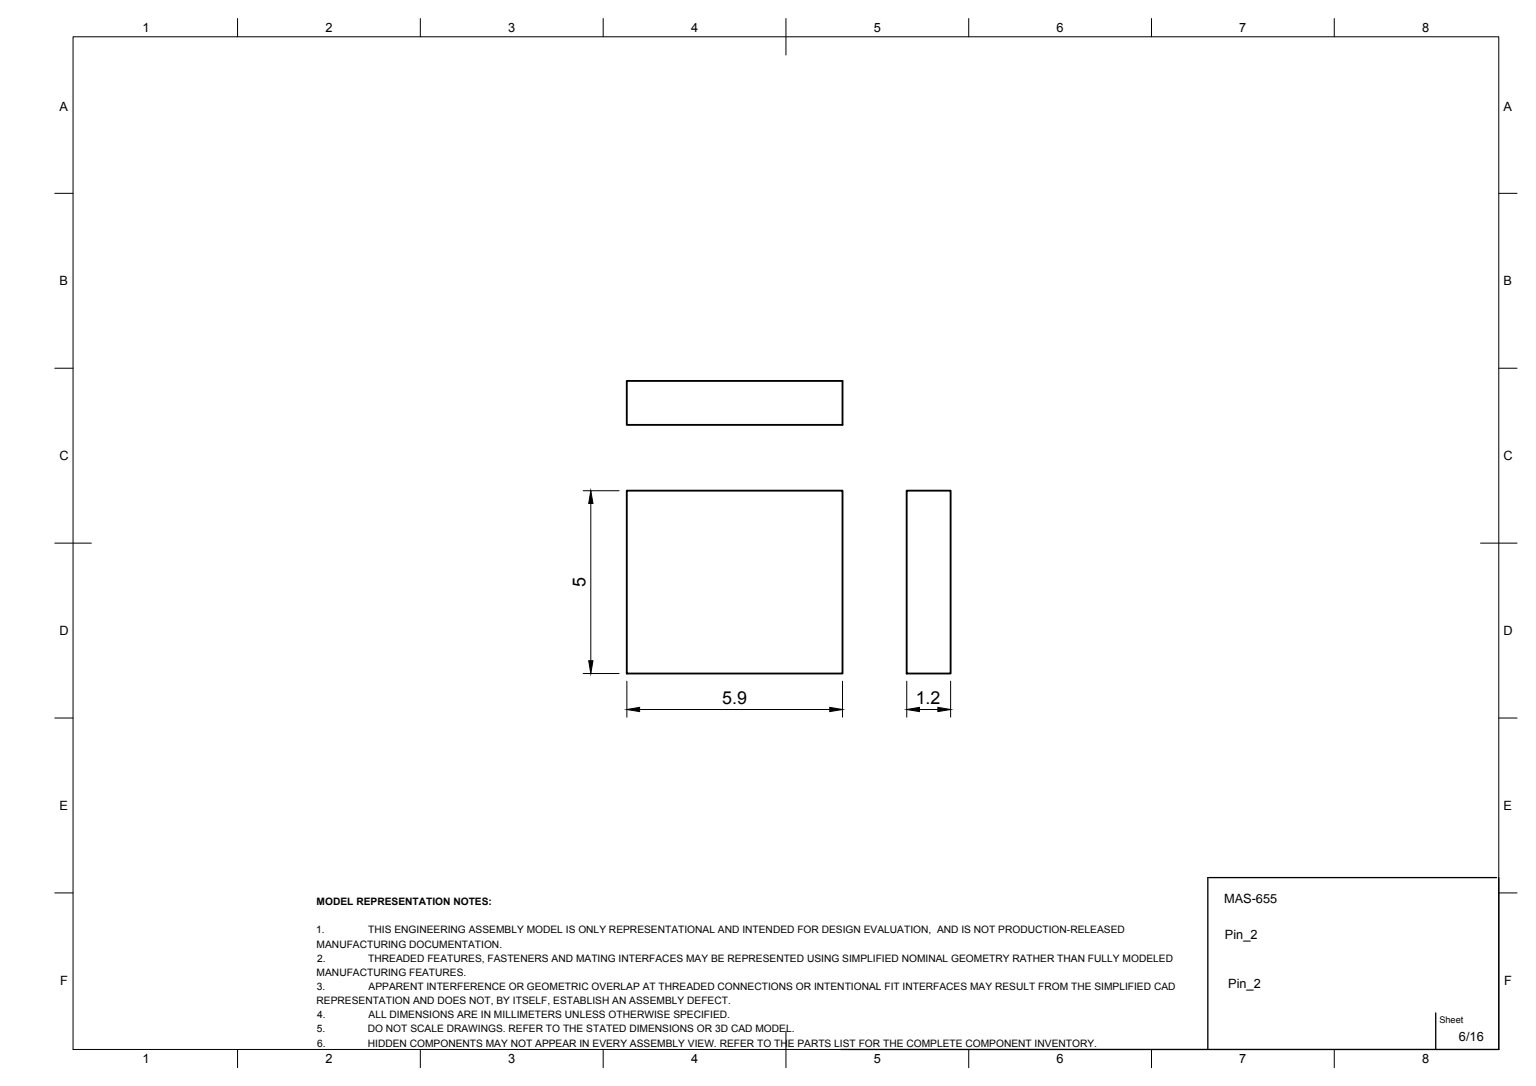
ISO-10303-21;
HEADER;
FILE_DESCRIPTION((''),'2;1');
FILE_NAME('Pin_2.step','2026-10-09T11:34:15-07:00',(''),(''),'','','');
FILE_SCHEMA (('AUTOMOTIVE_DESIGN { 1 0 10303 214 3 1 1 }'));
ENDSEC;
DATA;
#10=MECHANICAL_DESIGN_GEOMETRIC_PRESENTATION_REPRESENTATION('',(#633),#117170);
#591=SHAPE_REPRESENTATION_RELATIONSHIP('SRR','None',#117246,#612) ;
#612=ADVANCED_BREP_SHAPE_REPRESENTATION('',(#654),#117154) ;
#633=STYLED_ITEM('',(#117355),#654) ;
#654=MANIFOLD_SOLID_BREP('Body1',#49062) ;
#2476=PLANE('',#51975) ;
#2477=PLANE('',#51976) ;
#2478=PLANE('',#51977) ;
#2479=PLANE('',#51978) ;
#2480=PLANE('',#51979) ;
#2481=PLANE('',#51980) ;
#4253=LINE('',#87449,#7467) ;
#4254=LINE('',#87451,#7468) ;
#4255=LINE('',#87453,#7469) ;
#4256=LINE('',#87454,#7470) ;
#4257=LINE('',#87457,#7471) ;
#4258=LINE('',#87459,#7472) ;
#4259=LINE('',#87460,#7473) ;
#4260=LINE('',#87463,#7474) ;
#4261=LINE('',#87465,#7475) ;
#4262=LINE('',#87466,#7476) ;
#4263=LINE('',#87468,#7477) ;
#4264=LINE('',#87469,#7478) ;
#7467=VECTOR('',#61650,10.) ;
#7468=VECTOR('',#61651,10.) ;
#7469=VECTOR('',#61652,10.) ;
#7470=VECTOR('',#61653,10.) ;
#7471=VECTOR('',#61656,10.) ;
#7472=VECTOR('',#61657,10.) ;
#7473=VECTOR('',#61658,10.) ;
#7474=VECTOR('',#61661,10.) ;
#7475=VECTOR('',#61662,10.) ;
#7476=VECTOR('',#61663,10.) ;
#7477=VECTOR('',#61666,10.) ;
#7478=VECTOR('',#61667,10.) ;
#12097=FACE_OUTER_BOUND('',#15248,.T.) ;
#12098=FACE_OUTER_BOUND('',#15249,.T.) ;
#12099=FACE_OUTER_BOUND('',#15250,.T.) ;
#12100=FACE_OUTER_BOUND('',#15251,.T.) ;
#12101=FACE_OUTER_BOUND('',#15252,.T.) ;
#12102=FACE_OUTER_BOUND('',#15253,.T.) ;
#15248=EDGE_LOOP('',(#37250,#37251,#37252,#37253)) ;
#15249=EDGE_LOOP('',(#37254,#37255,#37256,#37257)) ;
#15250=EDGE_LOOP('',(#37258,#37259,#37260,#37261)) ;
#15251=EDGE_LOOP('',(#37262,#37263,#37264,#37265)) ;
#15252=EDGE_LOOP('',(#37266,#37267,#37268,#37269)) ;
#15253=EDGE_LOOP('',(#37270,#37271,#37272,#37273)) ;
#21368=VERTEX_POINT('',#87447) ;
#21369=VERTEX_POINT('',#87448) ;
#21370=VERTEX_POINT('',#87450) ;
#21371=VERTEX_POINT('',#87452) ;
#21372=VERTEX_POINT('',#87456) ;
#21373=VERTEX_POINT('',#87458) ;
#21374=VERTEX_POINT('',#87462) ;
#21375=VERTEX_POINT('',#87464) ;
#26903=EDGE_CURVE('',#21368,#21369,#4253,.T.) ;
#26904=EDGE_CURVE('',#21369,#21370,#4254,.T.) ;
#26905=EDGE_CURVE('',#21371,#21370,#4255,.T.) ;
#26906=EDGE_CURVE('',#21368,#21371,#4256,.T.) ;
#26907=EDGE_CURVE('',#21372,#21368,#4257,.T.) ;
#26908=EDGE_CURVE('',#21373,#21371,#4258,.T.) ;
#26909=EDGE_CURVE('',#21372,#21373,#4259,.T.) ;
#26910=EDGE_CURVE('',#21374,#21372,#4260,.T.) ;
#26911=EDGE_CURVE('',#21375,#21373,#4261,.T.) ;
#26912=EDGE_CURVE('',#21374,#21375,#4262,.T.) ;
#26913=EDGE_CURVE('',#21369,#21374,#4263,.T.) ;
#26914=EDGE_CURVE('',#21370,#21375,#4264,.T.) ;
#37250=ORIENTED_EDGE('',*,*,#26903,.T.) ;
#37251=ORIENTED_EDGE('',*,*,#26904,.T.) ;
#37252=ORIENTED_EDGE('',*,*,#26905,.F.) ;
#37253=ORIENTED_EDGE('',*,*,#26906,.F.) ;
#37254=ORIENTED_EDGE('',*,*,#26907,.T.) ;
#37255=ORIENTED_EDGE('',*,*,#26906,.T.) ;
#37256=ORIENTED_EDGE('',*,*,#26908,.F.) ;
#37257=ORIENTED_EDGE('',*,*,#26909,.F.) ;
#37258=ORIENTED_EDGE('',*,*,#26910,.T.) ;
#37259=ORIENTED_EDGE('',*,*,#26909,.T.) ;
#37260=ORIENTED_EDGE('',*,*,#26911,.F.) ;
#37261=ORIENTED_EDGE('',*,*,#26912,.F.) ;
#37262=ORIENTED_EDGE('',*,*,#26913,.T.) ;
#37263=ORIENTED_EDGE('',*,*,#26912,.T.) ;
#37264=ORIENTED_EDGE('',*,*,#26914,.F.) ;
#37265=ORIENTED_EDGE('',*,*,#26904,.F.) ;
#37266=ORIENTED_EDGE('',*,*,#26914,.T.) ;
#37267=ORIENTED_EDGE('',*,*,#26911,.T.) ;
#37268=ORIENTED_EDGE('',*,*,#26908,.T.) ;
#37269=ORIENTED_EDGE('',*,*,#26905,.T.) ;
#37270=ORIENTED_EDGE('',*,*,#26913,.F.) ;
#37271=ORIENTED_EDGE('',*,*,#26903,.F.) ;
#37272=ORIENTED_EDGE('',*,*,#26907,.F.) ;
#37273=ORIENTED_EDGE('',*,*,#26910,.F.) ;
#47315=ADVANCED_FACE('',(#12097),#2476,.T.) ;
#47316=ADVANCED_FACE('',(#12098),#2477,.T.) ;
#47317=ADVANCED_FACE('',(#12099),#2478,.T.) ;
#47318=ADVANCED_FACE('',(#12100),#2479,.T.) ;
#47319=ADVANCED_FACE('',(#12101),#2480,.T.) ;
#47320=ADVANCED_FACE('',(#12102),#2481,.F.) ;
#49062=CLOSED_SHELL('',(#47315,#47316,#47317,#47318,#47319,#47320)) ;
#51974=AXIS2_PLACEMENT_3D('',#87445,#61646,#61647) ;
#51975=AXIS2_PLACEMENT_3D('',#87446,#61648,#61649) ;
#51976=AXIS2_PLACEMENT_3D('',#87455,#61654,#61655) ;
#51977=AXIS2_PLACEMENT_3D('',#87461,#61659,#61660) ;
#51978=AXIS2_PLACEMENT_3D('',#87467,#61664,#61665) ;
#51979=AXIS2_PLACEMENT_3D('',#87470,#61668,#61669) ;
#51980=AXIS2_PLACEMENT_3D('',#87471,#61670,#61671) ;
#61646=DIRECTION('axis',(0.,0.,1.)) ;
#61647=DIRECTION('refdir',(1.,0.,0.)) ;
#61648=DIRECTION('center_axis',(0.,-1.,0.)) ;
#61649=DIRECTION('ref_axis',(-1.,0.,-2.52374105052742E-18)) ;
#61650=DIRECTION('',(-1.,0.,-2.52374105052742E-18)) ;
#61651=DIRECTION('',(0.,0.,-1.)) ;
#61652=DIRECTION('',(-1.,0.,-2.52374105052742E-18)) ;
#61653=DIRECTION('',(0.,0.,-1.)) ;
#61654=DIRECTION('center_axis',(1.,1.41426179436738E-51,0.)) ;
#61655=DIRECTION('ref_axis',(1.41426179436738E-51,-1.,-5.60383084497445E-34)) ;
#61656=DIRECTION('',(1.41426179436738E-51,-1.,-5.60383084497445E-34)) ;
#61657=DIRECTION('',(1.41426179436738E-51,-1.,-5.60383084497445E-34)) ;
#61658=DIRECTION('',(0.,0.,-1.)) ;
#61659=DIRECTION('center_axis',(0.,1.,0.)) ;
#61660=DIRECTION('ref_axis',(1.,0.,2.52374105052742E-18)) ;
#61661=DIRECTION('',(1.,0.,2.52374105052742E-18)) ;
#61662=DIRECTION('',(1.,0.,2.52374105052742E-18)) ;
#61663=DIRECTION('',(0.,0.,-1.)) ;
#61664=DIRECTION('center_axis',(-1.,-1.41426179436738E-51,0.)) ;
#61665=DIRECTION('ref_axis',(-1.41426179436738E-51,1.,5.60383084497445E-34)) ;
#61666=DIRECTION('',(-1.41426179436738E-51,1.,5.60383084497445E-34)) ;
#61667=DIRECTION('',(-1.41426179436738E-51,1.,5.60383084497445E-34)) ;
#61668=DIRECTION('center_axis',(0.,0.,-1.)) ;
#61669=DIRECTION('ref_axis',(-1.,0.,0.)) ;
#61670=DIRECTION('center_axis',(2.52374105052742E-18,5.60383084497445E-34,
-1.)) ;
#61671=DIRECTION('ref_axis',(1.,3.40207761657885E-68,2.52374105052742E-18)) ;
#87445=CARTESIAN_POINT('',(0.,0.,0.)) ;
#87446=CARTESIAN_POINT('Origin',(34.2,257.9,30.7213203435596)) ;
#87447=CARTESIAN_POINT('',(34.2,257.9,30.7213203435596)) ;
#87448=CARTESIAN_POINT('',(29.2,257.9,30.7213203435596)) ;
#87449=CARTESIAN_POINT('',(34.2,257.9,30.7213203435596)) ;
#87450=CARTESIAN_POINT('',(29.2,257.9,29.5213203435596)) ;
#87451=CARTESIAN_POINT('',(29.2,257.9,30.7213203435596)) ;
#87452=CARTESIAN_POINT('',(34.2,257.9,29.5213203435596)) ;
#87453=CARTESIAN_POINT('',(34.2,257.9,29.5213203435596)) ;
#87454=CARTESIAN_POINT('',(34.2,257.9,30.7213203435596)) ;
#87455=CARTESIAN_POINT('Origin',(34.2,263.8,30.7213203435596)) ;
#87456=CARTESIAN_POINT('',(34.2,263.8,30.7213203435596)) ;
#87457=CARTESIAN_POINT('',(34.2,263.8,30.7213203435596)) ;
#87458=CARTESIAN_POINT('',(34.2,263.8,29.5213203435596)) ;
#87459=CARTESIAN_POINT('',(34.2,263.8,29.5213203435596)) ;
#87460=CARTESIAN_POINT('',(34.2,263.8,30.7213203435596)) ;
#87461=CARTESIAN_POINT('Origin',(29.2,263.8,30.7213203435596)) ;
#87462=CARTESIAN_POINT('',(29.2,263.8,30.7213203435596)) ;
#87463=CARTESIAN_POINT('',(29.2,263.8,30.7213203435596)) ;
#87464=CARTESIAN_POINT('',(29.2,263.8,29.5213203435596)) ;
#87465=CARTESIAN_POINT('',(29.2,263.8,29.5213203435596)) ;
#87466=CARTESIAN_POINT('',(29.2,263.8,30.7213203435596)) ;
#87467=CARTESIAN_POINT('Origin',(29.2,257.9,30.7213203435596)) ;
#87468=CARTESIAN_POINT('',(29.2,257.9,30.7213203435596)) ;
#87469=CARTESIAN_POINT('',(29.2,257.9,29.5213203435596)) ;
#87470=CARTESIAN_POINT('Origin',(31.7,260.85,29.5213203435596)) ;
#87471=CARTESIAN_POINT('Origin',(31.7,260.85,30.7213203435596)) ;
#117131=UNCERTAINTY_MEASURE_WITH_UNIT(LENGTH_MEASURE(0.01),#117171,
'DISTANCE_ACCURACY_VALUE',
'Maximum model space distance between geometric entities at asserted c
onnectivities') ;
#117147=UNCERTAINTY_MEASURE_WITH_UNIT(LENGTH_MEASURE(0.01),#117171,
'DISTANCE_ACCURACY_VALUE',
'Maximum model space distance between geometric entities at asserted c
onnectivities') ;
#117154=(
GEOMETRIC_REPRESENTATION_CONTEXT(3)
GLOBAL_UNCERTAINTY_ASSIGNED_CONTEXT((#117131))
GLOBAL_UNIT_ASSIGNED_CONTEXT((#117171,#117173,#117174))
REPRESENTATION_CONTEXT('','3D')
) ;
#117170=(
GEOMETRIC_REPRESENTATION_CONTEXT(3)
GLOBAL_UNCERTAINTY_ASSIGNED_CONTEXT((#117147))
GLOBAL_UNIT_ASSIGNED_CONTEXT((#117171,#117173,#117174))
REPRESENTATION_CONTEXT('','3D')
) ;
#117171=(
LENGTH_UNIT()
NAMED_UNIT(*)
SI_UNIT(.MILLI.,.METRE.)
) ;
#117173=(
NAMED_UNIT(*)
PLANE_ANGLE_UNIT()
SI_UNIT($,.RADIAN.)
) ;
#117174=(
NAMED_UNIT(*)
SI_UNIT($,.STERADIAN.)
SOLID_ANGLE_UNIT()
) ;
#117181=SHAPE_DEFINITION_REPRESENTATION(#117203,#117246) ;
#117203=PRODUCT_DEFINITION_SHAPE('',$,#117269) ;
#117246=SHAPE_REPRESENTATION('',(#51974),#117154) ;
#117262=PRODUCT_DEFINITION_CONTEXT('part definition',#117330,'design') ;
#117269=PRODUCT_DEFINITION('Pin_2','Pin_2',#117291,#117262) ;
#117291=PRODUCT_DEFINITION_FORMATION('',$,#117338) ;
#117330=APPLICATION_CONTEXT(
'Core Data for Automotive Mechanical Design Process') ;
#117331=PRODUCT_CONTEXT('part definition',#117330,'mechanical') ;
#117338=PRODUCT('Pin_2','Pin_2',$,(#117331)) ;
#117355=PRESENTATION_STYLE_ASSIGNMENT((#117357)) ;
#117357=SURFACE_STYLE_USAGE(.BOTH.,#117359) ;
#117359=SURFACE_SIDE_STYLE('',(#117361)) ;
#117361=SURFACE_STYLE_FILL_AREA(#117363) ;
#117363=FILL_AREA_STYLE('Opaque(160,160,160)',(#117365)) ;
#117365=FILL_AREA_STYLE_COLOUR('Opaque(160,160,160)',#117367) ;
#117367=COLOUR_RGB('Opaque(160,160,160)', 0.09019608, 0.27058824, 0.51372549) ;
ENDSEC;
END-ISO-10303-21;
